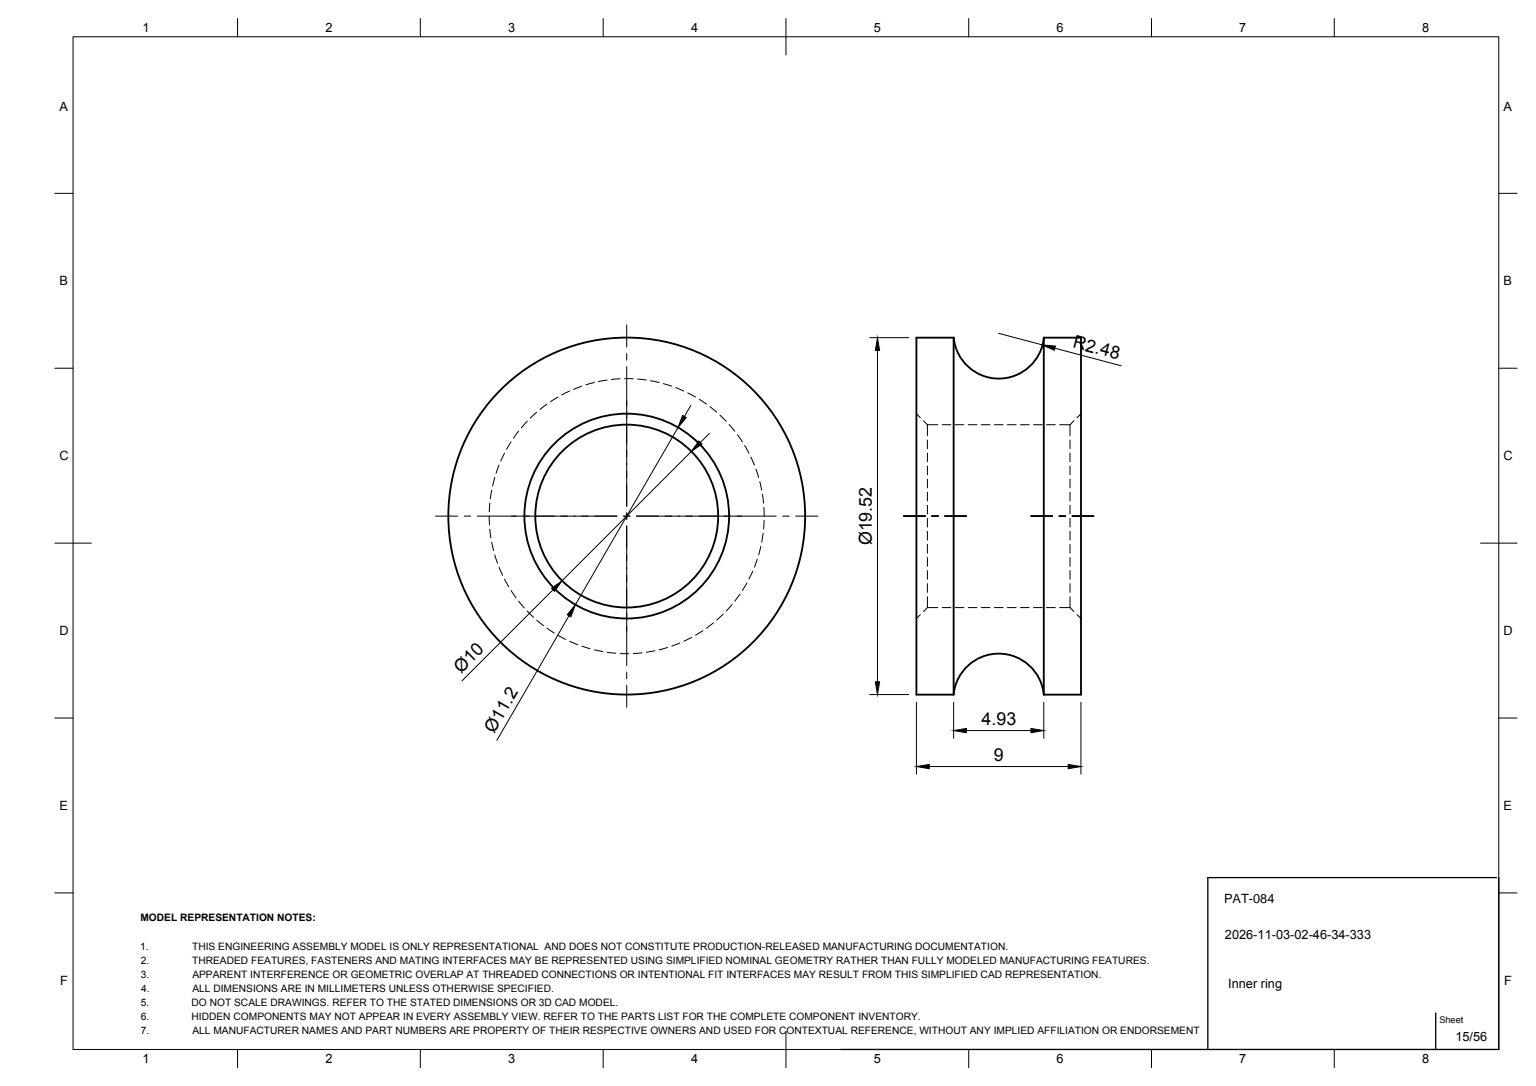
ISO-10303-21;
HEADER;
/* Generated by software containing ST-Developer
 * from STEP Tools, Inc. (www.steptools.com) 
 */

FILE_DESCRIPTION(
/* description */ ('Quick-return (Whitworth) mechanism'),
/* implementation_level */ '2;1');

FILE_NAME(
/* name */ 'Inner ring.step',
/* time_stamp */ '2026-10-28T03:25:57-07:00',
/* author */ (''),
/* organization */ (''),
/* preprocessor_version */ 'ST-DEVELOPER v20.2',
/* originating_system */ 'Autodesk Translation Framework v15.17.0.0',
/* authorisation */ '');

FILE_SCHEMA (('AUTOMOTIVE_DESIGN { 1 0 10303 214 3 1 1 }'));
ENDSEC;

DATA;
#10=MECHANICAL_DESIGN_GEOMETRIC_PRESENTATION_REPRESENTATION('',(#498),#14878);
#349=CONICAL_SURFACE('',#8721,0.53,0.785398163397448);
#350=CONICAL_SURFACE('',#8728,0.53,0.785398163397448);
#364=TOROIDAL_SURFACE('',#8710,1.,0.247676);
#410=SHAPE_REPRESENTATION_RELATIONSHIP('SRR','None',#15079,#454);
#454=ADVANCED_BREP_SHAPE_REPRESENTATION('',(#550),#14836);
#498=STYLED_ITEM('',(#15406),#550);
#550=MANIFOLD_SOLID_BREP('Body1',#7852);
#693=FACE_BOUND('',#1770,.T.);
#694=FACE_BOUND('',#1773,.T.);
#856=PLANE('',#8723);
#857=PLANE('',#8726);
#1197=FACE_OUTER_BOUND('',#1765,.T.);
#1198=FACE_OUTER_BOUND('',#1766,.T.);
#1199=FACE_OUTER_BOUND('',#1767,.T.);
#1200=FACE_OUTER_BOUND('',#1768,.T.);
#1201=FACE_OUTER_BOUND('',#1769,.T.);
#1202=FACE_OUTER_BOUND('',#1771,.T.);
#1203=FACE_OUTER_BOUND('',#1772,.T.);
#1204=FACE_OUTER_BOUND('',#1774,.T.);
#1765=EDGE_LOOP('',(#5918,#5919,#5920,#5921,#5922,#5923));
#1766=EDGE_LOOP('',(#5924,#5925,#5926,#5927,#5928));
#1767=EDGE_LOOP('',(#5929,#5930,#5931,#5932));
#1768=EDGE_LOOP('',(#5933,#5934,#5935,#5936));
#1769=EDGE_LOOP('',(#5937));
#1770=EDGE_LOOP('',(#5938));
#1771=EDGE_LOOP('',(#5939,#5940,#5941,#5942,#5943));
#1772=EDGE_LOOP('',(#5944));
#1773=EDGE_LOOP('',(#5945));
#1774=EDGE_LOOP('',(#5946,#5947,#5948,#5949));
#2326=LINE('',#12804,#2849);
#2327=LINE('',#12810,#2850);
#2328=LINE('',#12814,#2851);
#2329=LINE('',#12820,#2852);
#2330=LINE('',#12825,#2853);
#2849=VECTOR('',#10219,0.976185);
#2850=VECTOR('',#10226,0.5);
#2851=VECTOR('',#10231,0.53);
#2852=VECTOR('',#10240,0.976185);
#2853=VECTOR('',#10247,0.53);
#3380=CIRCLE('',#8711,0.976185);
#3381=CIRCLE('',#8712,0.976185);
#3382=CIRCLE('',#8713,0.247676);
#3383=CIRCLE('',#8714,0.976185);
#3384=CIRCLE('',#8715,0.976185);
#3385=CIRCLE('',#8717,0.976185);
#3386=CIRCLE('',#8719,0.5);
#3387=CIRCLE('',#8720,0.5);
#3388=CIRCLE('',#8722,0.56);
#3389=CIRCLE('',#8725,0.976185);
#3390=CIRCLE('',#8727,0.56);
#3851=VERTEX_POINT('',#12793);
#3852=VERTEX_POINT('',#12794);
#3853=VERTEX_POINT('',#12797);
#3854=VERTEX_POINT('',#12799);
#3855=VERTEX_POINT('',#12803);
#3856=VERTEX_POINT('',#12807);
#3857=VERTEX_POINT('',#12809);
#3858=VERTEX_POINT('',#12813);
#3859=VERTEX_POINT('',#12818);
#3860=VERTEX_POINT('',#12822);
#4616=EDGE_CURVE('',#3851,#3852,#3380,.T.);
#4617=EDGE_CURVE('',#3852,#3851,#3381,.T.);
#4618=EDGE_CURVE('',#3852,#3853,#3382,.T.);
#4619=EDGE_CURVE('',#3854,#3853,#3383,.T.);
#4620=EDGE_CURVE('',#3853,#3854,#3384,.T.);
#4621=EDGE_CURVE('',#3854,#3855,#2326,.T.);
#4622=EDGE_CURVE('',#3855,#3855,#3385,.T.);
#4623=EDGE_CURVE('',#3856,#3856,#3386,.T.);
#4624=EDGE_CURVE('',#3856,#3857,#2327,.T.);
#4625=EDGE_CURVE('',#3857,#3857,#3387,.T.);
#4626=EDGE_CURVE('',#3857,#3858,#2328,.T.);
#4627=EDGE_CURVE('',#3858,#3858,#3388,.T.);
#4628=EDGE_CURVE('',#3859,#3859,#3389,.T.);
#4629=EDGE_CURVE('',#3859,#3851,#2329,.T.);
#4630=EDGE_CURVE('',#3860,#3860,#3390,.T.);
#4631=EDGE_CURVE('',#3860,#3856,#2330,.T.);
#5918=ORIENTED_EDGE('',*,*,#4616,.F.);
#5919=ORIENTED_EDGE('',*,*,#4617,.F.);
#5920=ORIENTED_EDGE('',*,*,#4618,.T.);
#5921=ORIENTED_EDGE('',*,*,#4619,.F.);
#5922=ORIENTED_EDGE('',*,*,#4620,.F.);
#5923=ORIENTED_EDGE('',*,*,#4618,.F.);
#5924=ORIENTED_EDGE('',*,*,#4619,.T.);
#5925=ORIENTED_EDGE('',*,*,#4620,.T.);
#5926=ORIENTED_EDGE('',*,*,#4621,.T.);
#5927=ORIENTED_EDGE('',*,*,#4622,.T.);
#5928=ORIENTED_EDGE('',*,*,#4621,.F.);
#5929=ORIENTED_EDGE('',*,*,#4623,.T.);
#5930=ORIENTED_EDGE('',*,*,#4624,.T.);
#5931=ORIENTED_EDGE('',*,*,#4625,.F.);
#5932=ORIENTED_EDGE('',*,*,#4624,.F.);
#5933=ORIENTED_EDGE('',*,*,#4625,.T.);
#5934=ORIENTED_EDGE('',*,*,#4626,.T.);
#5935=ORIENTED_EDGE('',*,*,#4627,.F.);
#5936=ORIENTED_EDGE('',*,*,#4626,.F.);
#5937=ORIENTED_EDGE('',*,*,#4622,.F.);
#5938=ORIENTED_EDGE('',*,*,#4627,.T.);
#5939=ORIENTED_EDGE('',*,*,#4628,.F.);
#5940=ORIENTED_EDGE('',*,*,#4629,.T.);
#5941=ORIENTED_EDGE('',*,*,#4616,.T.);
#5942=ORIENTED_EDGE('',*,*,#4617,.T.);
#5943=ORIENTED_EDGE('',*,*,#4629,.F.);
#5944=ORIENTED_EDGE('',*,*,#4628,.T.);
#5945=ORIENTED_EDGE('',*,*,#4630,.F.);
#5946=ORIENTED_EDGE('',*,*,#4630,.T.);
#5947=ORIENTED_EDGE('',*,*,#4631,.T.);
#5948=ORIENTED_EDGE('',*,*,#4623,.F.);
#5949=ORIENTED_EDGE('',*,*,#4631,.F.);
#7286=CYLINDRICAL_SURFACE('',#8716,0.976185);
#7287=CYLINDRICAL_SURFACE('',#8718,0.5);
#7288=CYLINDRICAL_SURFACE('',#8724,0.976185);
#7528=ADVANCED_FACE('',(#1197),#364,.F.);
#7529=ADVANCED_FACE('',(#1198),#7286,.T.);
#7530=ADVANCED_FACE('',(#1199),#7287,.F.);
#7531=ADVANCED_FACE('',(#1200),#349,.F.);
#7532=ADVANCED_FACE('',(#1201,#693),#856,.T.);
#7533=ADVANCED_FACE('',(#1202),#7288,.T.);
#7534=ADVANCED_FACE('',(#1203,#694),#857,.T.);
#7535=ADVANCED_FACE('',(#1204),#350,.F.);
#7852=CLOSED_SHELL('',(#7528,#7529,#7530,#7531,#7532,#7533,#7534,#7535));
#8709=AXIS2_PLACEMENT_3D('',#12791,#10203,#10204);
#8710=AXIS2_PLACEMENT_3D('',#12792,#10205,#10206);
#8711=AXIS2_PLACEMENT_3D('',#12795,#10207,#10208);
#8712=AXIS2_PLACEMENT_3D('',#12796,#10209,#10210);
#8713=AXIS2_PLACEMENT_3D('',#12798,#10211,#10212);
#8714=AXIS2_PLACEMENT_3D('',#12800,#10213,#10214);
#8715=AXIS2_PLACEMENT_3D('',#12801,#10215,#10216);
#8716=AXIS2_PLACEMENT_3D('',#12802,#10217,#10218);
#8717=AXIS2_PLACEMENT_3D('',#12805,#10220,#10221);
#8718=AXIS2_PLACEMENT_3D('',#12806,#10222,#10223);
#8719=AXIS2_PLACEMENT_3D('',#12808,#10224,#10225);
#8720=AXIS2_PLACEMENT_3D('',#12811,#10227,#10228);
#8721=AXIS2_PLACEMENT_3D('',#12812,#10229,#10230);
#8722=AXIS2_PLACEMENT_3D('',#12815,#10232,#10233);
#8723=AXIS2_PLACEMENT_3D('',#12816,#10234,#10235);
#8724=AXIS2_PLACEMENT_3D('',#12817,#10236,#10237);
#8725=AXIS2_PLACEMENT_3D('',#12819,#10238,#10239);
#8726=AXIS2_PLACEMENT_3D('',#12821,#10241,#10242);
#8727=AXIS2_PLACEMENT_3D('',#12823,#10243,#10244);
#8728=AXIS2_PLACEMENT_3D('',#12824,#10245,#10246);
#10203=DIRECTION('axis',(0.,0.,1.));
#10204=DIRECTION('refdir',(1.,0.,0.));
#10205=DIRECTION('center_axis',(0.,-1.,0.));
#10206=DIRECTION('ref_axis',(0.,0.,-1.));
#10207=DIRECTION('center_axis',(0.,-1.,0.));
#10208=DIRECTION('ref_axis',(1.,0.,0.));
#10209=DIRECTION('center_axis',(0.,-1.,0.));
#10210=DIRECTION('ref_axis',(1.,0.,0.));
#10211=DIRECTION('center_axis',(1.,0.,1.22464679914735E-16));
#10212=DIRECTION('ref_axis',(-1.22464679914735E-16,0.,1.));
#10213=DIRECTION('center_axis',(0.,1.,0.));
#10214=DIRECTION('ref_axis',(1.,0.,0.));
#10215=DIRECTION('center_axis',(0.,1.,0.));
#10216=DIRECTION('ref_axis',(1.,0.,0.));
#10217=DIRECTION('center_axis',(0.,-1.,0.));
#10218=DIRECTION('ref_axis',(1.,0.,0.));
#10219=DIRECTION('',(0.,1.,0.));
#10220=DIRECTION('center_axis',(0.,-1.,0.));
#10221=DIRECTION('ref_axis',(1.,0.,0.));
#10222=DIRECTION('center_axis',(0.,-1.,0.));
#10223=DIRECTION('ref_axis',(1.,0.,0.));
#10224=DIRECTION('center_axis',(0.,-1.,0.));
#10225=DIRECTION('ref_axis',(1.,0.,0.));
#10226=DIRECTION('',(0.,1.,0.));
#10227=DIRECTION('center_axis',(0.,-1.,0.));
#10228=DIRECTION('ref_axis',(1.,0.,0.));
#10229=DIRECTION('center_axis',(0.,1.,0.));
#10230=DIRECTION('ref_axis',(1.,0.,0.));
#10231=DIRECTION('',(-0.707106781186547,0.707106781186548,-8.65956056235493E-17));
#10232=DIRECTION('center_axis',(0.,-1.,0.));
#10233=DIRECTION('ref_axis',(1.,0.,0.));
#10234=DIRECTION('center_axis',(0.,1.,0.));
#10235=DIRECTION('ref_axis',(0.,0.,1.));
#10236=DIRECTION('center_axis',(0.,-1.,0.));
#10237=DIRECTION('ref_axis',(1.,0.,0.));
#10238=DIRECTION('center_axis',(0.,-1.,0.));
#10239=DIRECTION('ref_axis',(1.,0.,0.));
#10240=DIRECTION('',(0.,1.,0.));
#10241=DIRECTION('center_axis',(0.,-1.,0.));
#10242=DIRECTION('ref_axis',(0.,0.,-1.));
#10243=DIRECTION('center_axis',(0.,-1.,0.));
#10244=DIRECTION('ref_axis',(1.,0.,0.));
#10245=DIRECTION('center_axis',(0.,-1.,0.));
#10246=DIRECTION('ref_axis',(1.,0.,0.));
#10247=DIRECTION('',(0.707106781186547,0.707106781186548,8.65956056235493E-17));
#12791=CARTESIAN_POINT('',(0.,0.,0.));
#12792=CARTESIAN_POINT('Origin',(0.,0.,0.));
#12793=CARTESIAN_POINT('',(-0.976185,-0.246528389340863,-1.19548183562566E-16));
#12794=CARTESIAN_POINT('',(-1.19548183562566E-16,-0.246528389340863,0.976185));
#12795=CARTESIAN_POINT('Origin',(0.,-0.246528389340863,0.));
#12796=CARTESIAN_POINT('Origin',(0.,-0.246528389340863,0.));
#12797=CARTESIAN_POINT('',(-1.19548183562566E-16,0.246528389340863,0.976185));
#12798=CARTESIAN_POINT('Origin',(-1.22464679914735E-16,0.,1.));
#12799=CARTESIAN_POINT('',(-0.976185,0.246528389340863,1.19548183562566E-16));
#12800=CARTESIAN_POINT('Origin',(0.,0.246528389340863,0.));
#12801=CARTESIAN_POINT('Origin',(0.,0.246528389340863,0.));
#12802=CARTESIAN_POINT('Origin',(0.,0.,0.));
#12803=CARTESIAN_POINT('',(-0.976185,0.45,-1.19548183562566E-16));
#12804=CARTESIAN_POINT('',(-0.976185,0.,-1.19548183562566E-16));
#12805=CARTESIAN_POINT('Origin',(0.,0.45,0.));
#12806=CARTESIAN_POINT('Origin',(0.,0.,0.));
#12807=CARTESIAN_POINT('',(-0.5,-0.39,-6.12323399573677E-17));
#12808=CARTESIAN_POINT('Origin',(0.,-0.39,0.));
#12809=CARTESIAN_POINT('',(-0.5,0.39,-6.12323399573677E-17));
#12810=CARTESIAN_POINT('',(-0.5,0.,-6.12323399573677E-17));
#12811=CARTESIAN_POINT('Origin',(0.,0.39,0.));
#12812=CARTESIAN_POINT('Origin',(0.,0.42,0.));
#12813=CARTESIAN_POINT('',(-0.56,0.45,-6.85802207522518E-17));
#12814=CARTESIAN_POINT('',(-0.53,0.42,-6.49062803548097E-17));
#12815=CARTESIAN_POINT('Origin',(0.,0.45,0.));
#12816=CARTESIAN_POINT('Origin',(0.976185,0.45,0.));
#12817=CARTESIAN_POINT('Origin',(0.,0.,0.));
#12818=CARTESIAN_POINT('',(-0.976185,-0.45,-1.19548183562566E-16));
#12819=CARTESIAN_POINT('Origin',(0.,-0.45,0.));
#12820=CARTESIAN_POINT('',(-0.976185,0.,-1.19548183562566E-16));
#12821=CARTESIAN_POINT('Origin',(0.56,-0.45,0.));
#12822=CARTESIAN_POINT('',(-0.56,-0.45,-6.85802207522518E-17));
#12823=CARTESIAN_POINT('Origin',(0.,-0.45,0.));
#12824=CARTESIAN_POINT('Origin',(0.,-0.42,0.));
#12825=CARTESIAN_POINT('',(-0.53,-0.42,-6.49062803548097E-17));
#14782=UNCERTAINTY_MEASURE_WITH_UNIT(LENGTH_MEASURE(0.001),#14879,
'DISTANCE_ACCURACY_VALUE',
'Maximum model space distance between geometric entities at asserted c
onnectivities');
#14824=UNCERTAINTY_MEASURE_WITH_UNIT(LENGTH_MEASURE(0.001),#14879,
'DISTANCE_ACCURACY_VALUE',
'Maximum model space distance between geometric entities at asserted c
onnectivities');
#14836=(
GEOMETRIC_REPRESENTATION_CONTEXT(3)
GLOBAL_UNCERTAINTY_ASSIGNED_CONTEXT((#14782))
GLOBAL_UNIT_ASSIGNED_CONTEXT((#14879,#14881,#14882))
REPRESENTATION_CONTEXT('','3D')
);
#14878=(
GEOMETRIC_REPRESENTATION_CONTEXT(3)
GLOBAL_UNCERTAINTY_ASSIGNED_CONTEXT((#14824))
GLOBAL_UNIT_ASSIGNED_CONTEXT((#14879,#14881,#14882))
REPRESENTATION_CONTEXT('','3D')
);
#14879=(
LENGTH_UNIT()
NAMED_UNIT(*)
SI_UNIT(.CENTI.,.METRE.)
);
#14881=(
NAMED_UNIT(*)
PLANE_ANGLE_UNIT()
SI_UNIT($,.RADIAN.)
);
#14882=(
NAMED_UNIT(*)
SI_UNIT($,.STERADIAN.)
SOLID_ANGLE_UNIT()
);
#14894=SHAPE_DEFINITION_REPRESENTATION(#14947,#15079);
#14947=PRODUCT_DEFINITION_SHAPE('',$,#15133);
#15079=SHAPE_REPRESENTATION('',(#8709),#14836);
#15121=PRODUCT_DEFINITION_CONTEXT('part definition',#15282,'design');
#15133=PRODUCT_DEFINITION('Inner ring','Inner ring',#15186,#15121);
#15186=PRODUCT_DEFINITION_FORMATION('',$,#15295);
#15282=APPLICATION_CONTEXT(
'Core Data for Automotive Mechanical Design Process');
#15283=PRODUCT_CONTEXT('part definition',#15282,'mechanical');
#15295=PRODUCT('Inner ring','Inner ring','Inner ring',(#15283));
#15400=COLOUR_RGB('Grey',0.48,0.52,0.57);
#15401=FILL_AREA_STYLE_COLOUR('',#15400);
#15402=FILL_AREA_STYLE('',(#15401));
#15403=SURFACE_STYLE_FILL_AREA(#15402);
#15404=SURFACE_SIDE_STYLE('',(#15403));
#15405=SURFACE_STYLE_USAGE(.BOTH.,#15404);
#15406=PRESENTATION_STYLE_ASSIGNMENT((#15405));
ENDSEC;
END-ISO-10303-21;
